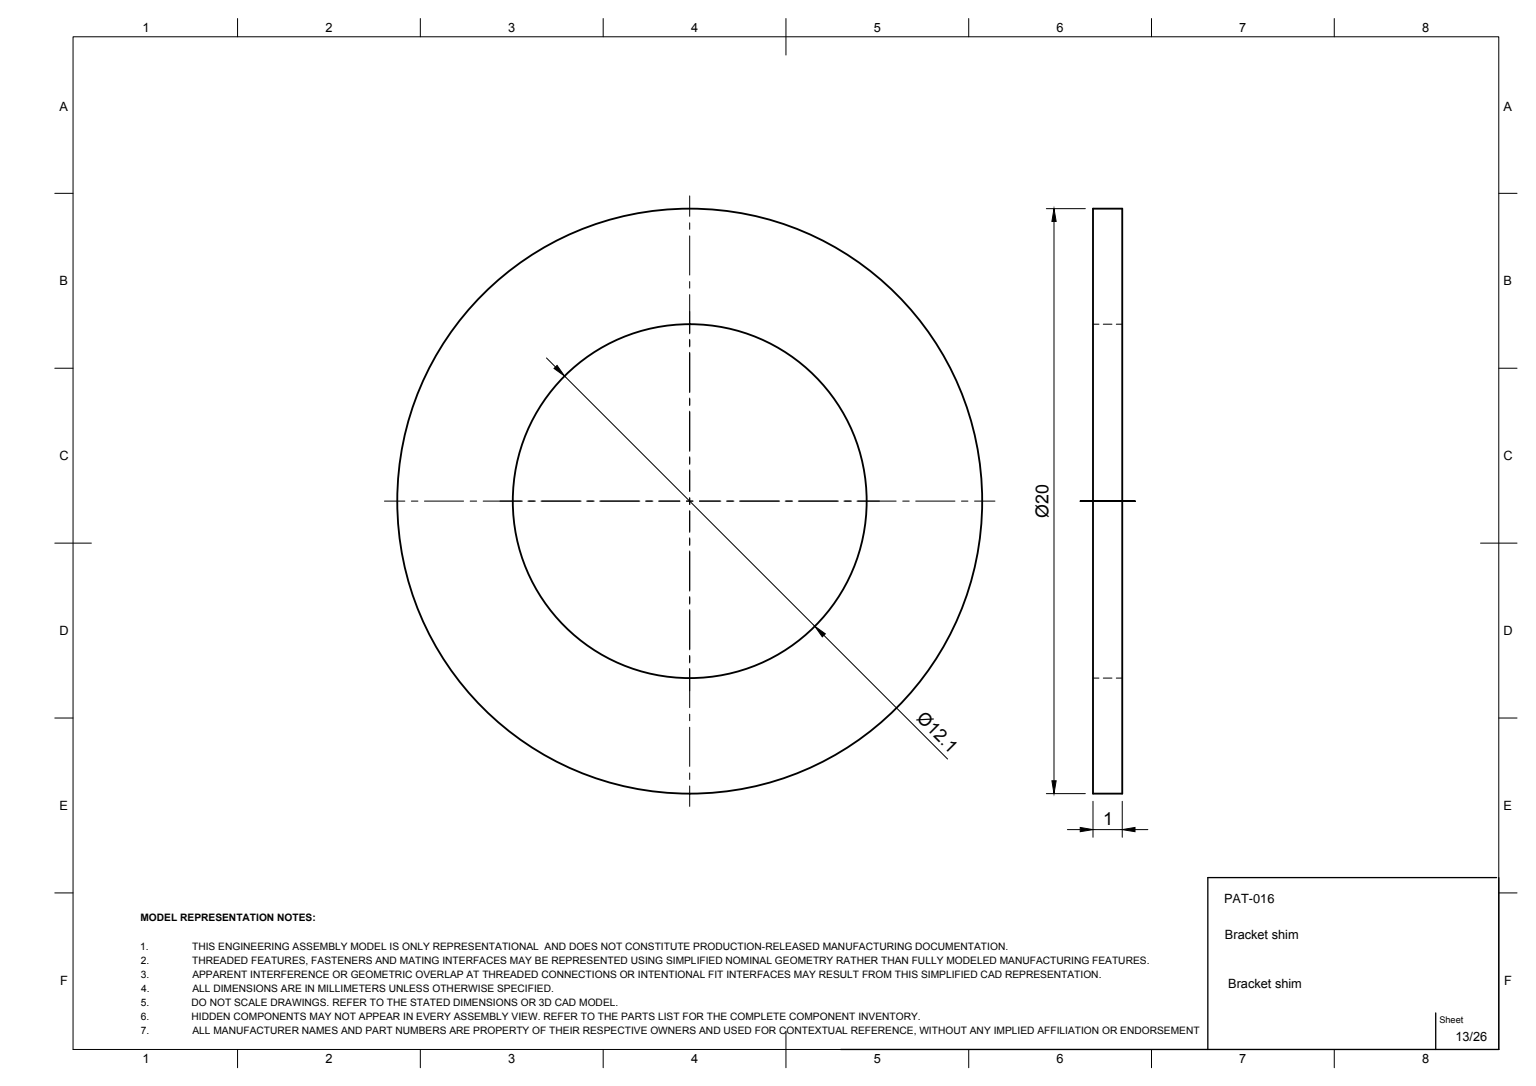
ISO-10303-21;
HEADER;
/* Generated by software containing ST-Developer
 * from STEP Tools, Inc. (www.steptools.com) 
 */

FILE_DESCRIPTION(
/* description */ ('Bracket-mounted idler roller'),
/* implementation_level */ '2;1');

FILE_NAME(
/* name */ 'Bracket shim.step',
/* time_stamp */ '2026-10-28T03:26:42-07:00',
/* author */ (''),
/* organization */ (''),
/* preprocessor_version */ 'ST-DEVELOPER v20.2',
/* originating_system */ 'Autodesk Translation Framework v15.17.0.0',
/* authorisation */ '');

FILE_SCHEMA (('AUTOMOTIVE_DESIGN { 1 0 10303 214 3 1 1 }'));
ENDSEC;

DATA;
#10=MECHANICAL_DESIGN_GEOMETRIC_PRESENTATION_REPRESENTATION('',(#290),#6241);
#248=SHAPE_REPRESENTATION_RELATIONSHIP('SRR','None',#6352,#269);
#269=ADVANCED_BREP_SHAPE_REPRESENTATION('',(#318),#6228);
#290=STYLED_ITEM('',(#6517),#318);
#318=MANIFOLD_SOLID_BREP('Body1',#3193);
#371=FACE_BOUND('',#832,.T.);
#372=FACE_BOUND('',#834,.T.);
#476=PLANE('',#3604);
#477=PLANE('',#3605);
#603=FACE_OUTER_BOUND('',#829,.T.);
#604=FACE_OUTER_BOUND('',#830,.T.);
#605=FACE_OUTER_BOUND('',#831,.T.);
#606=FACE_OUTER_BOUND('',#833,.T.);
#829=EDGE_LOOP('',(#2508,#2509,#2510,#2511));
#830=EDGE_LOOP('',(#2512,#2513,#2514,#2515));
#831=EDGE_LOOP('',(#2516));
#832=EDGE_LOOP('',(#2517));
#833=EDGE_LOOP('',(#2518));
#834=EDGE_LOOP('',(#2519));
#1097=LINE('',#5338,#1279);
#1098=LINE('',#5344,#1280);
#1279=VECTOR('',#4314,0.605);
#1280=VECTOR('',#4321,1.);
#1396=CIRCLE('',#3599,0.605);
#1397=CIRCLE('',#3600,0.605);
#1398=CIRCLE('',#3602,1.);
#1399=CIRCLE('',#3603,1.);
#1637=VERTEX_POINT('',#5335);
#1638=VERTEX_POINT('',#5337);
#1639=VERTEX_POINT('',#5341);
#1640=VERTEX_POINT('',#5343);
#1956=EDGE_CURVE('',#1637,#1637,#1396,.T.);
#1957=EDGE_CURVE('',#1637,#1638,#1097,.T.);
#1958=EDGE_CURVE('',#1638,#1638,#1397,.T.);
#1959=EDGE_CURVE('',#1639,#1639,#1398,.T.);
#1960=EDGE_CURVE('',#1639,#1640,#1098,.T.);
#1961=EDGE_CURVE('',#1640,#1640,#1399,.T.);
#2508=ORIENTED_EDGE('',*,*,#1956,.F.);
#2509=ORIENTED_EDGE('',*,*,#1957,.T.);
#2510=ORIENTED_EDGE('',*,*,#1958,.T.);
#2511=ORIENTED_EDGE('',*,*,#1957,.F.);
#2512=ORIENTED_EDGE('',*,*,#1959,.F.);
#2513=ORIENTED_EDGE('',*,*,#1960,.T.);
#2514=ORIENTED_EDGE('',*,*,#1961,.T.);
#2515=ORIENTED_EDGE('',*,*,#1960,.F.);
#2516=ORIENTED_EDGE('',*,*,#1959,.T.);
#2517=ORIENTED_EDGE('',*,*,#1956,.T.);
#2518=ORIENTED_EDGE('',*,*,#1961,.F.);
#2519=ORIENTED_EDGE('',*,*,#1958,.F.);
#2953=CYLINDRICAL_SURFACE('',#3598,0.605);
#2954=CYLINDRICAL_SURFACE('',#3601,1.);
#3078=ADVANCED_FACE('',(#603),#2953,.F.);
#3079=ADVANCED_FACE('',(#604),#2954,.T.);
#3080=ADVANCED_FACE('',(#605,#371),#476,.T.);
#3081=ADVANCED_FACE('',(#606,#372),#477,.F.);
#3193=CLOSED_SHELL('',(#3078,#3079,#3080,#3081));
#3597=AXIS2_PLACEMENT_3D('',#5333,#4308,#4309);
#3598=AXIS2_PLACEMENT_3D('',#5334,#4310,#4311);
#3599=AXIS2_PLACEMENT_3D('',#5336,#4312,#4313);
#3600=AXIS2_PLACEMENT_3D('',#5339,#4315,#4316);
#3601=AXIS2_PLACEMENT_3D('',#5340,#4317,#4318);
#3602=AXIS2_PLACEMENT_3D('',#5342,#4319,#4320);
#3603=AXIS2_PLACEMENT_3D('',#5345,#4322,#4323);
#3604=AXIS2_PLACEMENT_3D('',#5346,#4324,#4325);
#3605=AXIS2_PLACEMENT_3D('',#5347,#4326,#4327);
#4308=DIRECTION('axis',(0.,0.,1.));
#4309=DIRECTION('refdir',(1.,0.,0.));
#4310=DIRECTION('center_axis',(0.,1.,0.));
#4311=DIRECTION('ref_axis',(1.,0.,0.));
#4312=DIRECTION('center_axis',(0.,-1.,0.));
#4313=DIRECTION('ref_axis',(1.,0.,0.));
#4314=DIRECTION('',(0.,-1.,0.));
#4315=DIRECTION('center_axis',(0.,-1.,0.));
#4316=DIRECTION('ref_axis',(1.,0.,0.));
#4317=DIRECTION('center_axis',(0.,1.,0.));
#4318=DIRECTION('ref_axis',(1.,0.,0.));
#4319=DIRECTION('center_axis',(0.,1.,0.));
#4320=DIRECTION('ref_axis',(1.,0.,0.));
#4321=DIRECTION('',(0.,-1.,0.));
#4322=DIRECTION('center_axis',(0.,1.,0.));
#4323=DIRECTION('ref_axis',(1.,0.,0.));
#4324=DIRECTION('center_axis',(0.,1.,0.));
#4325=DIRECTION('ref_axis',(1.,0.,0.));
#4326=DIRECTION('center_axis',(0.,1.,0.));
#4327=DIRECTION('ref_axis',(1.,0.,0.));
#5333=CARTESIAN_POINT('',(0.,0.,0.));
#5334=CARTESIAN_POINT('Origin',(0.,-2.5,4.5));
#5335=CARTESIAN_POINT('',(-0.605,-2.4,4.5));
#5336=CARTESIAN_POINT('Origin',(0.,-2.4,4.5));
#5337=CARTESIAN_POINT('',(-0.605,-2.5,4.5));
#5338=CARTESIAN_POINT('',(-0.605,-2.5,4.5));
#5339=CARTESIAN_POINT('Origin',(0.,-2.5,4.5));
#5340=CARTESIAN_POINT('Origin',(0.,-2.5,4.5));
#5341=CARTESIAN_POINT('',(-1.,-2.4,4.5));
#5342=CARTESIAN_POINT('Origin',(0.,-2.4,4.5));
#5343=CARTESIAN_POINT('',(-1.,-2.5,4.5));
#5344=CARTESIAN_POINT('',(-1.,-2.5,4.5));
#5345=CARTESIAN_POINT('Origin',(0.,-2.5,4.5));
#5346=CARTESIAN_POINT('Origin',(0.,-2.4,4.5));
#5347=CARTESIAN_POINT('Origin',(0.,-2.5,4.5));
#6202=UNCERTAINTY_MEASURE_WITH_UNIT(LENGTH_MEASURE(0.001),#6242,
'DISTANCE_ACCURACY_VALUE',
'Maximum model space distance between geometric entities at asserted c
onnectivities');
#6215=UNCERTAINTY_MEASURE_WITH_UNIT(LENGTH_MEASURE(0.001),#6242,
'DISTANCE_ACCURACY_VALUE',
'Maximum model space distance between geometric entities at asserted c
onnectivities');
#6228=(
GEOMETRIC_REPRESENTATION_CONTEXT(3)
GLOBAL_UNCERTAINTY_ASSIGNED_CONTEXT((#6202))
GLOBAL_UNIT_ASSIGNED_CONTEXT((#6242,#6244,#6245))
REPRESENTATION_CONTEXT('','3D')
);
#6241=(
GEOMETRIC_REPRESENTATION_CONTEXT(3)
GLOBAL_UNCERTAINTY_ASSIGNED_CONTEXT((#6215))
GLOBAL_UNIT_ASSIGNED_CONTEXT((#6242,#6244,#6245))
REPRESENTATION_CONTEXT('','3D')
);
#6242=(
LENGTH_UNIT()
NAMED_UNIT(*)
SI_UNIT(.CENTI.,.METRE.)
);
#6244=(
NAMED_UNIT(*)
PLANE_ANGLE_UNIT()
SI_UNIT($,.RADIAN.)
);
#6245=(
NAMED_UNIT(*)
SI_UNIT($,.STERADIAN.)
SOLID_ANGLE_UNIT()
);
#6258=SHAPE_DEFINITION_REPRESENTATION(#6283,#6352);
#6283=PRODUCT_DEFINITION_SHAPE('',$,#6378);
#6352=SHAPE_REPRESENTATION('',(#3597),#6228);
#6365=PRODUCT_DEFINITION_CONTEXT('part definition',#6442,'design');
#6378=PRODUCT_DEFINITION('Bracket shim','Bracket shim',#6403,#6365);
#6403=PRODUCT_DEFINITION_FORMATION('',$,#6456);
#6442=APPLICATION_CONTEXT(
'Core Data for Automotive Mechanical Design Process');
#6443=PRODUCT_CONTEXT('part definition',#6442,'mechanical');
#6456=PRODUCT('Bracket shim','Bracket shim','Bracket shim',(#6443));
#6511=COLOUR_RGB('Dark Blue',0.08,0.2,0.34);
#6512=FILL_AREA_STYLE_COLOUR('',#6511);
#6513=FILL_AREA_STYLE('',(#6512));
#6514=SURFACE_STYLE_FILL_AREA(#6513);
#6515=SURFACE_SIDE_STYLE('',(#6514));
#6516=SURFACE_STYLE_USAGE(.BOTH.,#6515);
#6517=PRESENTATION_STYLE_ASSIGNMENT((#6516));
ENDSEC;
END-ISO-10303-21;
